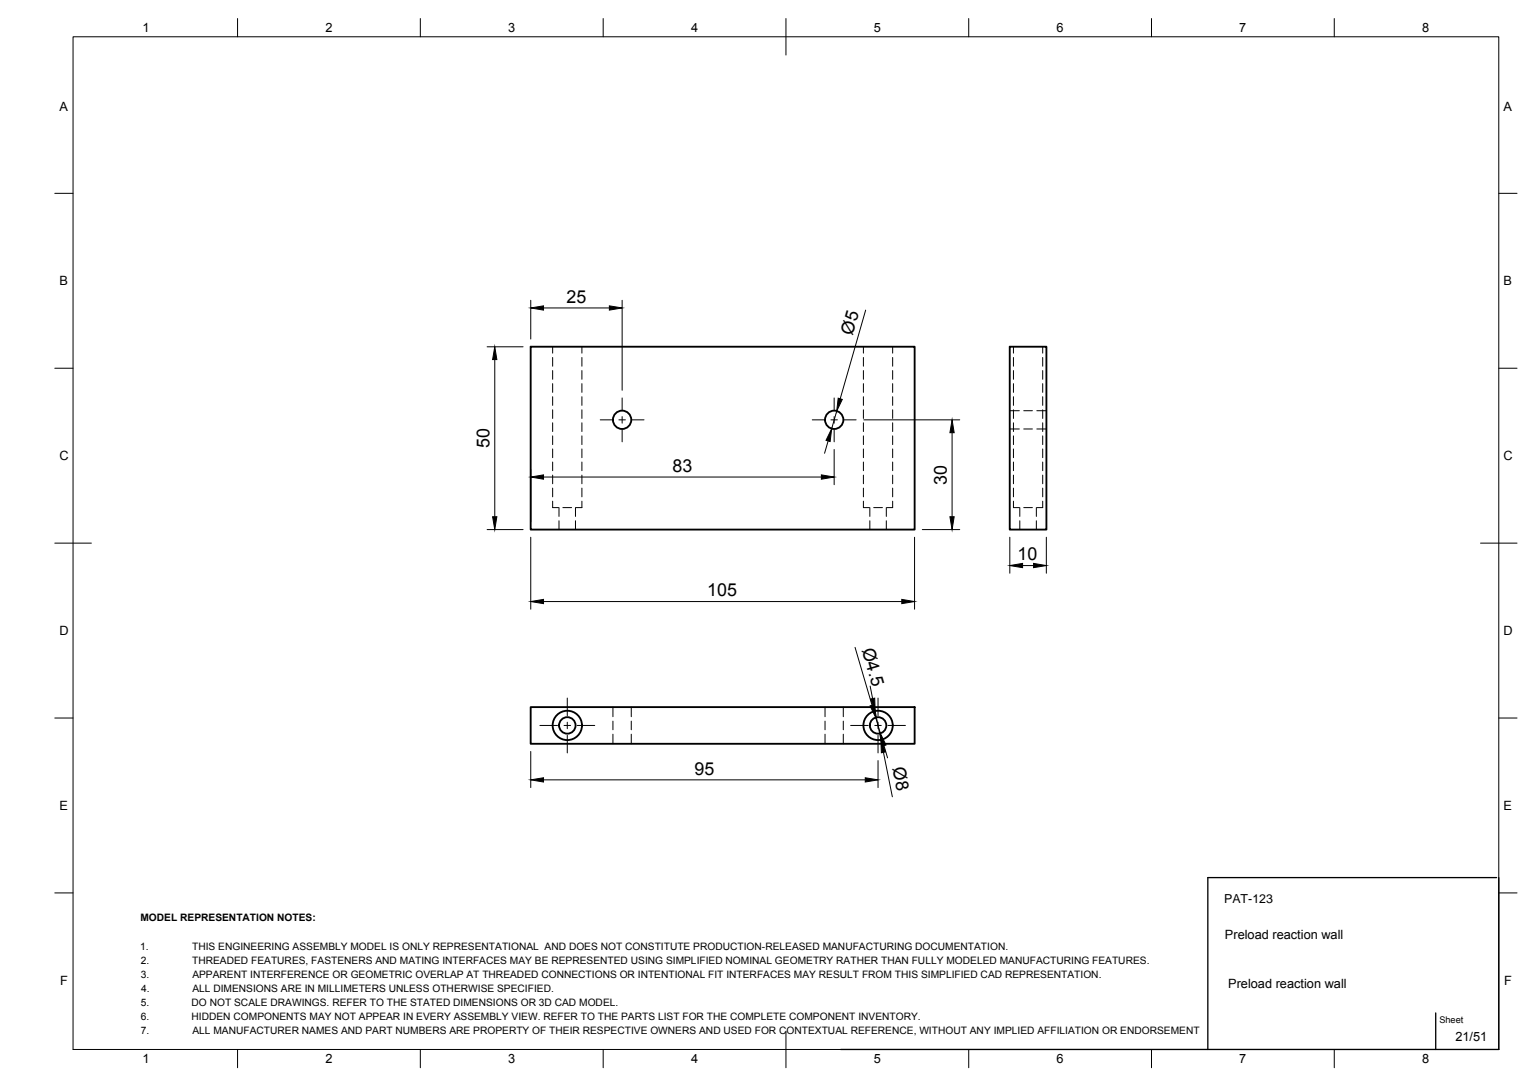
ISO-10303-21;
HEADER;
/* Generated by software containing ST-Developer
 * from STEP Tools, Inc. (www.steptools.com) 
 */

FILE_DESCRIPTION(
/* description */ ('Worm-less right-angle friction wheel drive'),
/* implementation_level */ '2;1');

FILE_NAME(
/* name */ 'Preload reaction wall.step',
/* time_stamp */ '2026-10-28T03:22:36-07:00',
/* author */ (''),
/* organization */ (''),
/* preprocessor_version */ 'ST-DEVELOPER v20.2',
/* originating_system */ 'Autodesk Translation Framework v15.17.0.0',
/* authorisation */ '');

FILE_SCHEMA (('AUTOMOTIVE_DESIGN { 1 0 10303 214 3 1 1 }'));
ENDSEC;

DATA;
#10=MECHANICAL_DESIGN_GEOMETRIC_PRESENTATION_REPRESENTATION('',(#627),#17046);
#533=SHAPE_REPRESENTATION_RELATIONSHIP('SRR','None',#17276,#580);
#580=ADVANCED_BREP_SHAPE_REPRESENTATION('',(#681),#17012);
#627=STYLED_ITEM('',(#17605),#681);
#681=MANIFOLD_SOLID_BREP('Body1',#8182);
#895=FACE_BOUND('',#2060,.T.);
#896=FACE_BOUND('',#2064,.T.);
#897=FACE_BOUND('',#2067,.T.);
#898=FACE_BOUND('',#2068,.T.);
#899=FACE_BOUND('',#2071,.T.);
#900=FACE_BOUND('',#2072,.T.);
#901=FACE_BOUND('',#2075,.T.);
#902=FACE_BOUND('',#2076,.T.);
#903=FACE_BOUND('',#2078,.T.);
#904=FACE_BOUND('',#2079,.T.);
#1048=PLANE('',#9184);
#1049=PLANE('',#9191);
#1050=PLANE('',#9195);
#1051=PLANE('',#9196);
#1052=PLANE('',#9197);
#1053=PLANE('',#9198);
#1054=PLANE('',#9199);
#1055=PLANE('',#9200);
#1410=FACE_OUTER_BOUND('',#2056,.T.);
#1411=FACE_OUTER_BOUND('',#2057,.T.);
#1412=FACE_OUTER_BOUND('',#2058,.T.);
#1413=FACE_OUTER_BOUND('',#2059,.T.);
#1414=FACE_OUTER_BOUND('',#2061,.T.);
#1415=FACE_OUTER_BOUND('',#2062,.T.);
#1416=FACE_OUTER_BOUND('',#2063,.T.);
#1417=FACE_OUTER_BOUND('',#2065,.T.);
#1418=FACE_OUTER_BOUND('',#2066,.T.);
#1419=FACE_OUTER_BOUND('',#2069,.T.);
#1420=FACE_OUTER_BOUND('',#2070,.T.);
#1421=FACE_OUTER_BOUND('',#2073,.T.);
#1422=FACE_OUTER_BOUND('',#2074,.T.);
#1423=FACE_OUTER_BOUND('',#2077,.T.);
#2056=EDGE_LOOP('',(#6506,#6507,#6508,#6509));
#2057=EDGE_LOOP('',(#6510,#6511,#6512,#6513));
#2058=EDGE_LOOP('',(#6514,#6515,#6516,#6517));
#2059=EDGE_LOOP('',(#6518));
#2060=EDGE_LOOP('',(#6519));
#2061=EDGE_LOOP('',(#6520,#6521,#6522,#6523));
#2062=EDGE_LOOP('',(#6524,#6525,#6526,#6527));
#2063=EDGE_LOOP('',(#6528));
#2064=EDGE_LOOP('',(#6529));
#2065=EDGE_LOOP('',(#6530,#6531,#6532,#6533));
#2066=EDGE_LOOP('',(#6534,#6535,#6536,#6537));
#2067=EDGE_LOOP('',(#6538));
#2068=EDGE_LOOP('',(#6539));
#2069=EDGE_LOOP('',(#6540,#6541,#6542,#6543));
#2070=EDGE_LOOP('',(#6544,#6545,#6546,#6547));
#2071=EDGE_LOOP('',(#6548));
#2072=EDGE_LOOP('',(#6549));
#2073=EDGE_LOOP('',(#6550,#6551,#6552,#6553));
#2074=EDGE_LOOP('',(#6554,#6555,#6556,#6557));
#2075=EDGE_LOOP('',(#6558));
#2076=EDGE_LOOP('',(#6559));
#2077=EDGE_LOOP('',(#6560,#6561,#6562,#6563));
#2078=EDGE_LOOP('',(#6564));
#2079=EDGE_LOOP('',(#6565));
#2651=LINE('',#13410,#3191);
#2652=LINE('',#13416,#3192);
#2653=LINE('',#13422,#3193);
#2654=LINE('',#13430,#3194);
#2655=LINE('',#13435,#3195);
#2656=LINE('',#13443,#3196);
#2657=LINE('',#13447,#3197);
#2658=LINE('',#13449,#3198);
#2659=LINE('',#13451,#3199);
#2660=LINE('',#13452,#3200);
#2661=LINE('',#13455,#3201);
#2662=LINE('',#13457,#3202);
#2663=LINE('',#13458,#3203);
#2664=LINE('',#13461,#3204);
#2665=LINE('',#13463,#3205);
#2666=LINE('',#13464,#3206);
#2667=LINE('',#13466,#3207);
#2668=LINE('',#13467,#3208);
#3191=VECTOR('',#10917,0.25);
#3192=VECTOR('',#10924,0.25);
#3193=VECTOR('',#10931,0.4);
#3194=VECTOR('',#10942,0.225);
#3195=VECTOR('',#10947,0.4);
#3196=VECTOR('',#10958,0.225);
#3197=VECTOR('',#10961,1.);
#3198=VECTOR('',#10962,1.);
#3199=VECTOR('',#10963,1.);
#3200=VECTOR('',#10964,1.);
#3201=VECTOR('',#10967,1.);
#3202=VECTOR('',#10968,1.);
#3203=VECTOR('',#10969,1.);
#3204=VECTOR('',#10972,1.);
#3205=VECTOR('',#10973,1.);
#3206=VECTOR('',#10974,1.);
#3207=VECTOR('',#10977,1.);
#3208=VECTOR('',#10978,1.);
#3669=CIRCLE('',#9176,0.25);
#3670=CIRCLE('',#9177,0.25);
#3671=CIRCLE('',#9179,0.25);
#3672=CIRCLE('',#9180,0.25);
#3673=CIRCLE('',#9182,0.4);
#3674=CIRCLE('',#9183,0.4);
#3675=CIRCLE('',#9185,0.225);
#3676=CIRCLE('',#9187,0.225);
#3677=CIRCLE('',#9189,0.4);
#3678=CIRCLE('',#9190,0.4);
#3679=CIRCLE('',#9192,0.225);
#3680=CIRCLE('',#9194,0.225);
#4193=VERTEX_POINT('',#13407);
#4194=VERTEX_POINT('',#13409);
#4195=VERTEX_POINT('',#13413);
#4196=VERTEX_POINT('',#13415);
#4197=VERTEX_POINT('',#13419);
#4198=VERTEX_POINT('',#13421);
#4199=VERTEX_POINT('',#13425);
#4200=VERTEX_POINT('',#13428);
#4201=VERTEX_POINT('',#13432);
#4202=VERTEX_POINT('',#13434);
#4203=VERTEX_POINT('',#13438);
#4204=VERTEX_POINT('',#13441);
#4205=VERTEX_POINT('',#13445);
#4206=VERTEX_POINT('',#13446);
#4207=VERTEX_POINT('',#13448);
#4208=VERTEX_POINT('',#13450);
#4209=VERTEX_POINT('',#13454);
#4210=VERTEX_POINT('',#13456);
#4211=VERTEX_POINT('',#13460);
#4212=VERTEX_POINT('',#13462);
#5022=EDGE_CURVE('',#4193,#4193,#3669,.T.);
#5023=EDGE_CURVE('',#4193,#4194,#2651,.T.);
#5024=EDGE_CURVE('',#4194,#4194,#3670,.T.);
#5025=EDGE_CURVE('',#4195,#4195,#3671,.T.);
#5026=EDGE_CURVE('',#4195,#4196,#2652,.T.);
#5027=EDGE_CURVE('',#4196,#4196,#3672,.T.);
#5028=EDGE_CURVE('',#4197,#4197,#3673,.T.);
#5029=EDGE_CURVE('',#4197,#4198,#2653,.T.);
#5030=EDGE_CURVE('',#4198,#4198,#3674,.T.);
#5031=EDGE_CURVE('',#4199,#4199,#3675,.T.);
#5032=EDGE_CURVE('',#4200,#4200,#3676,.T.);
#5033=EDGE_CURVE('',#4200,#4199,#2654,.T.);
#5034=EDGE_CURVE('',#4201,#4201,#3677,.T.);
#5035=EDGE_CURVE('',#4201,#4202,#2655,.T.);
#5036=EDGE_CURVE('',#4202,#4202,#3678,.T.);
#5037=EDGE_CURVE('',#4203,#4203,#3679,.T.);
#5038=EDGE_CURVE('',#4204,#4204,#3680,.T.);
#5039=EDGE_CURVE('',#4204,#4203,#2656,.T.);
#5040=EDGE_CURVE('',#4205,#4206,#2657,.T.);
#5041=EDGE_CURVE('',#4206,#4207,#2658,.T.);
#5042=EDGE_CURVE('',#4208,#4207,#2659,.T.);
#5043=EDGE_CURVE('',#4205,#4208,#2660,.T.);
#5044=EDGE_CURVE('',#4209,#4205,#2661,.T.);
#5045=EDGE_CURVE('',#4210,#4208,#2662,.T.);
#5046=EDGE_CURVE('',#4209,#4210,#2663,.T.);
#5047=EDGE_CURVE('',#4211,#4209,#2664,.T.);
#5048=EDGE_CURVE('',#4212,#4210,#2665,.T.);
#5049=EDGE_CURVE('',#4211,#4212,#2666,.T.);
#5050=EDGE_CURVE('',#4206,#4211,#2667,.T.);
#5051=EDGE_CURVE('',#4207,#4212,#2668,.T.);
#6506=ORIENTED_EDGE('',*,*,#5022,.F.);
#6507=ORIENTED_EDGE('',*,*,#5023,.T.);
#6508=ORIENTED_EDGE('',*,*,#5024,.F.);
#6509=ORIENTED_EDGE('',*,*,#5023,.F.);
#6510=ORIENTED_EDGE('',*,*,#5025,.F.);
#6511=ORIENTED_EDGE('',*,*,#5026,.T.);
#6512=ORIENTED_EDGE('',*,*,#5027,.F.);
#6513=ORIENTED_EDGE('',*,*,#5026,.F.);
#6514=ORIENTED_EDGE('',*,*,#5028,.F.);
#6515=ORIENTED_EDGE('',*,*,#5029,.T.);
#6516=ORIENTED_EDGE('',*,*,#5030,.F.);
#6517=ORIENTED_EDGE('',*,*,#5029,.F.);
#6518=ORIENTED_EDGE('',*,*,#5028,.T.);
#6519=ORIENTED_EDGE('',*,*,#5031,.F.);
#6520=ORIENTED_EDGE('',*,*,#5032,.F.);
#6521=ORIENTED_EDGE('',*,*,#5033,.T.);
#6522=ORIENTED_EDGE('',*,*,#5031,.T.);
#6523=ORIENTED_EDGE('',*,*,#5033,.F.);
#6524=ORIENTED_EDGE('',*,*,#5034,.F.);
#6525=ORIENTED_EDGE('',*,*,#5035,.T.);
#6526=ORIENTED_EDGE('',*,*,#5036,.F.);
#6527=ORIENTED_EDGE('',*,*,#5035,.F.);
#6528=ORIENTED_EDGE('',*,*,#5034,.T.);
#6529=ORIENTED_EDGE('',*,*,#5037,.F.);
#6530=ORIENTED_EDGE('',*,*,#5038,.F.);
#6531=ORIENTED_EDGE('',*,*,#5039,.T.);
#6532=ORIENTED_EDGE('',*,*,#5037,.T.);
#6533=ORIENTED_EDGE('',*,*,#5039,.F.);
#6534=ORIENTED_EDGE('',*,*,#5040,.T.);
#6535=ORIENTED_EDGE('',*,*,#5041,.T.);
#6536=ORIENTED_EDGE('',*,*,#5042,.F.);
#6537=ORIENTED_EDGE('',*,*,#5043,.F.);
#6538=ORIENTED_EDGE('',*,*,#5024,.T.);
#6539=ORIENTED_EDGE('',*,*,#5027,.T.);
#6540=ORIENTED_EDGE('',*,*,#5044,.T.);
#6541=ORIENTED_EDGE('',*,*,#5043,.T.);
#6542=ORIENTED_EDGE('',*,*,#5045,.F.);
#6543=ORIENTED_EDGE('',*,*,#5046,.F.);
#6544=ORIENTED_EDGE('',*,*,#5047,.T.);
#6545=ORIENTED_EDGE('',*,*,#5046,.T.);
#6546=ORIENTED_EDGE('',*,*,#5048,.F.);
#6547=ORIENTED_EDGE('',*,*,#5049,.F.);
#6548=ORIENTED_EDGE('',*,*,#5022,.T.);
#6549=ORIENTED_EDGE('',*,*,#5025,.T.);
#6550=ORIENTED_EDGE('',*,*,#5050,.T.);
#6551=ORIENTED_EDGE('',*,*,#5049,.T.);
#6552=ORIENTED_EDGE('',*,*,#5051,.F.);
#6553=ORIENTED_EDGE('',*,*,#5041,.F.);
#6554=ORIENTED_EDGE('',*,*,#5051,.T.);
#6555=ORIENTED_EDGE('',*,*,#5048,.T.);
#6556=ORIENTED_EDGE('',*,*,#5045,.T.);
#6557=ORIENTED_EDGE('',*,*,#5042,.T.);
#6558=ORIENTED_EDGE('',*,*,#5030,.T.);
#6559=ORIENTED_EDGE('',*,*,#5036,.T.);
#6560=ORIENTED_EDGE('',*,*,#5050,.F.);
#6561=ORIENTED_EDGE('',*,*,#5040,.F.);
#6562=ORIENTED_EDGE('',*,*,#5044,.F.);
#6563=ORIENTED_EDGE('',*,*,#5047,.F.);
#6564=ORIENTED_EDGE('',*,*,#5032,.T.);
#6565=ORIENTED_EDGE('',*,*,#5038,.T.);
#7636=CYLINDRICAL_SURFACE('',#9175,0.25);
#7637=CYLINDRICAL_SURFACE('',#9178,0.25);
#7638=CYLINDRICAL_SURFACE('',#9181,0.4);
#7639=CYLINDRICAL_SURFACE('',#9186,0.225);
#7640=CYLINDRICAL_SURFACE('',#9188,0.4);
#7641=CYLINDRICAL_SURFACE('',#9193,0.225);
#7902=ADVANCED_FACE('',(#1410),#7636,.F.);
#7903=ADVANCED_FACE('',(#1411),#7637,.F.);
#7904=ADVANCED_FACE('',(#1412),#7638,.F.);
#7905=ADVANCED_FACE('',(#1413,#895),#1048,.T.);
#7906=ADVANCED_FACE('',(#1414),#7639,.F.);
#7907=ADVANCED_FACE('',(#1415),#7640,.F.);
#7908=ADVANCED_FACE('',(#1416,#896),#1049,.T.);
#7909=ADVANCED_FACE('',(#1417),#7641,.F.);
#7910=ADVANCED_FACE('',(#1418,#897,#898),#1050,.T.);
#7911=ADVANCED_FACE('',(#1419),#1051,.T.);
#7912=ADVANCED_FACE('',(#1420,#899,#900),#1052,.T.);
#7913=ADVANCED_FACE('',(#1421),#1053,.T.);
#7914=ADVANCED_FACE('',(#1422,#901,#902),#1054,.T.);
#7915=ADVANCED_FACE('',(#1423,#903,#904),#1055,.F.);
#8182=CLOSED_SHELL('',(#7902,#7903,#7904,#7905,#7906,#7907,#7908,#7909,
#7910,#7911,#7912,#7913,#7914,#7915));
#9174=AXIS2_PLACEMENT_3D('',#13405,#10911,#10912);
#9175=AXIS2_PLACEMENT_3D('',#13406,#10913,#10914);
#9176=AXIS2_PLACEMENT_3D('',#13408,#10915,#10916);
#9177=AXIS2_PLACEMENT_3D('',#13411,#10918,#10919);
#9178=AXIS2_PLACEMENT_3D('',#13412,#10920,#10921);
#9179=AXIS2_PLACEMENT_3D('',#13414,#10922,#10923);
#9180=AXIS2_PLACEMENT_3D('',#13417,#10925,#10926);
#9181=AXIS2_PLACEMENT_3D('',#13418,#10927,#10928);
#9182=AXIS2_PLACEMENT_3D('',#13420,#10929,#10930);
#9183=AXIS2_PLACEMENT_3D('',#13423,#10932,#10933);
#9184=AXIS2_PLACEMENT_3D('',#13424,#10934,#10935);
#9185=AXIS2_PLACEMENT_3D('',#13426,#10936,#10937);
#9186=AXIS2_PLACEMENT_3D('',#13427,#10938,#10939);
#9187=AXIS2_PLACEMENT_3D('',#13429,#10940,#10941);
#9188=AXIS2_PLACEMENT_3D('',#13431,#10943,#10944);
#9189=AXIS2_PLACEMENT_3D('',#13433,#10945,#10946);
#9190=AXIS2_PLACEMENT_3D('',#13436,#10948,#10949);
#9191=AXIS2_PLACEMENT_3D('',#13437,#10950,#10951);
#9192=AXIS2_PLACEMENT_3D('',#13439,#10952,#10953);
#9193=AXIS2_PLACEMENT_3D('',#13440,#10954,#10955);
#9194=AXIS2_PLACEMENT_3D('',#13442,#10956,#10957);
#9195=AXIS2_PLACEMENT_3D('',#13444,#10959,#10960);
#9196=AXIS2_PLACEMENT_3D('',#13453,#10965,#10966);
#9197=AXIS2_PLACEMENT_3D('',#13459,#10970,#10971);
#9198=AXIS2_PLACEMENT_3D('',#13465,#10975,#10976);
#9199=AXIS2_PLACEMENT_3D('',#13468,#10979,#10980);
#9200=AXIS2_PLACEMENT_3D('',#13469,#10981,#10982);
#10911=DIRECTION('axis',(0.,0.,1.));
#10912=DIRECTION('refdir',(1.,0.,0.));
#10913=DIRECTION('center_axis',(0.,1.,0.));
#10914=DIRECTION('ref_axis',(1.,0.,0.));
#10915=DIRECTION('center_axis',(0.,1.,0.));
#10916=DIRECTION('ref_axis',(1.,0.,0.));
#10917=DIRECTION('',(0.,1.,0.));
#10918=DIRECTION('center_axis',(0.,-1.,0.));
#10919=DIRECTION('ref_axis',(1.,0.,0.));
#10920=DIRECTION('center_axis',(0.,1.,0.));
#10921=DIRECTION('ref_axis',(1.,0.,0.));
#10922=DIRECTION('center_axis',(0.,1.,0.));
#10923=DIRECTION('ref_axis',(1.,0.,0.));
#10924=DIRECTION('',(0.,1.,0.));
#10925=DIRECTION('center_axis',(0.,-1.,0.));
#10926=DIRECTION('ref_axis',(1.,0.,0.));
#10927=DIRECTION('center_axis',(0.,0.,1.));
#10928=DIRECTION('ref_axis',(1.,0.,0.));
#10929=DIRECTION('center_axis',(0.,0.,1.));
#10930=DIRECTION('ref_axis',(1.,0.,0.));
#10931=DIRECTION('',(0.,0.,1.));
#10932=DIRECTION('center_axis',(0.,0.,-1.));
#10933=DIRECTION('ref_axis',(1.,0.,0.));
#10934=DIRECTION('center_axis',(0.,0.,1.));
#10935=DIRECTION('ref_axis',(1.,0.,0.));
#10936=DIRECTION('center_axis',(0.,0.,1.));
#10937=DIRECTION('ref_axis',(1.,0.,0.));
#10938=DIRECTION('center_axis',(0.,0.,1.));
#10939=DIRECTION('ref_axis',(1.,0.,0.));
#10940=DIRECTION('center_axis',(0.,0.,1.));
#10941=DIRECTION('ref_axis',(1.,0.,0.));
#10942=DIRECTION('',(0.,0.,1.));
#10943=DIRECTION('center_axis',(0.,0.,1.));
#10944=DIRECTION('ref_axis',(1.,0.,0.));
#10945=DIRECTION('center_axis',(0.,0.,1.));
#10946=DIRECTION('ref_axis',(1.,0.,0.));
#10947=DIRECTION('',(0.,0.,1.));
#10948=DIRECTION('center_axis',(0.,0.,-1.));
#10949=DIRECTION('ref_axis',(1.,0.,0.));
#10950=DIRECTION('center_axis',(0.,0.,1.));
#10951=DIRECTION('ref_axis',(1.,0.,0.));
#10952=DIRECTION('center_axis',(0.,0.,1.));
#10953=DIRECTION('ref_axis',(1.,0.,0.));
#10954=DIRECTION('center_axis',(0.,0.,1.));
#10955=DIRECTION('ref_axis',(1.,0.,0.));
#10956=DIRECTION('center_axis',(0.,0.,1.));
#10957=DIRECTION('ref_axis',(1.,0.,0.));
#10958=DIRECTION('',(0.,0.,1.));
#10959=DIRECTION('center_axis',(0.,1.,0.));
#10960=DIRECTION('ref_axis',(-1.,0.,0.));
#10961=DIRECTION('',(-1.,0.,0.));
#10962=DIRECTION('',(0.,0.,1.));
#10963=DIRECTION('',(-1.,0.,0.));
#10964=DIRECTION('',(0.,0.,1.));
#10965=DIRECTION('center_axis',(1.,0.,0.));
#10966=DIRECTION('ref_axis',(0.,1.,0.));
#10967=DIRECTION('',(0.,1.,0.));
#10968=DIRECTION('',(0.,1.,0.));
#10969=DIRECTION('',(0.,0.,1.));
#10970=DIRECTION('center_axis',(0.,-1.,0.));
#10971=DIRECTION('ref_axis',(1.,0.,0.));
#10972=DIRECTION('',(1.,0.,0.));
#10973=DIRECTION('',(1.,0.,0.));
#10974=DIRECTION('',(0.,0.,1.));
#10975=DIRECTION('center_axis',(-1.,0.,0.));
#10976=DIRECTION('ref_axis',(0.,-1.,0.));
#10977=DIRECTION('',(0.,-1.,0.));
#10978=DIRECTION('',(0.,-1.,0.));
#10979=DIRECTION('center_axis',(0.,0.,1.));
#10980=DIRECTION('ref_axis',(1.,0.,0.));
#10981=DIRECTION('center_axis',(0.,0.,1.));
#10982=DIRECTION('ref_axis',(1.,0.,0.));
#13405=CARTESIAN_POINT('',(0.,0.,0.));
#13406=CARTESIAN_POINT('Origin',(5.5,7.9,4.));
#13407=CARTESIAN_POINT('',(5.25,8.,4.));
#13408=CARTESIAN_POINT('Origin',(5.5,8.,4.));
#13409=CARTESIAN_POINT('',(5.25,9.,4.));
#13410=CARTESIAN_POINT('',(5.25,7.9,4.));
#13411=CARTESIAN_POINT('Origin',(5.5,9.,4.));
#13412=CARTESIAN_POINT('Origin',(-0.3,7.9,4.));
#13413=CARTESIAN_POINT('',(-0.55,8.,4.));
#13414=CARTESIAN_POINT('Origin',(-0.3,8.,4.));
#13415=CARTESIAN_POINT('',(-0.55,9.,4.));
#13416=CARTESIAN_POINT('',(-0.55,7.9,4.));
#13417=CARTESIAN_POINT('Origin',(-0.3,9.,4.));
#13418=CARTESIAN_POINT('Origin',(7.,8.5,1.6));
#13419=CARTESIAN_POINT('',(6.6,8.5,1.6));
#13420=CARTESIAN_POINT('Origin',(7.,8.5,1.6));
#13421=CARTESIAN_POINT('',(6.6,8.5,6.));
#13422=CARTESIAN_POINT('',(6.6,8.5,1.6));
#13423=CARTESIAN_POINT('Origin',(7.,8.5,6.));
#13424=CARTESIAN_POINT('Origin',(7.,8.5,1.6));
#13425=CARTESIAN_POINT('',(6.775,8.5,1.6));
#13426=CARTESIAN_POINT('Origin',(7.,8.5,1.6));
#13427=CARTESIAN_POINT('Origin',(7.,8.5,0.9));
#13428=CARTESIAN_POINT('',(6.775,8.5,1.));
#13429=CARTESIAN_POINT('Origin',(7.,8.5,1.));
#13430=CARTESIAN_POINT('',(6.775,8.5,0.9));
#13431=CARTESIAN_POINT('Origin',(-1.5,8.5,1.6));
#13432=CARTESIAN_POINT('',(-1.9,8.5,1.6));
#13433=CARTESIAN_POINT('Origin',(-1.5,8.5,1.6));
#13434=CARTESIAN_POINT('',(-1.9,8.5,6.));
#13435=CARTESIAN_POINT('',(-1.9,8.5,1.6));
#13436=CARTESIAN_POINT('Origin',(-1.5,8.5,6.));
#13437=CARTESIAN_POINT('Origin',(-1.5,8.5,1.6));
#13438=CARTESIAN_POINT('',(-1.725,8.5,1.6));
#13439=CARTESIAN_POINT('Origin',(-1.5,8.5,1.6));
#13440=CARTESIAN_POINT('Origin',(-1.5,8.5,0.9));
#13441=CARTESIAN_POINT('',(-1.725,8.5,1.));
#13442=CARTESIAN_POINT('Origin',(-1.5,8.5,1.));
#13443=CARTESIAN_POINT('',(-1.725,8.5,0.9));
#13444=CARTESIAN_POINT('Origin',(8.,9.,1.));
#13445=CARTESIAN_POINT('',(8.,9.,1.));
#13446=CARTESIAN_POINT('',(-2.5,9.,1.));
#13447=CARTESIAN_POINT('',(8.,9.,1.));
#13448=CARTESIAN_POINT('',(-2.5,9.,6.));
#13449=CARTESIAN_POINT('',(-2.5,9.,1.));
#13450=CARTESIAN_POINT('',(8.,9.,6.));
#13451=CARTESIAN_POINT('',(8.,9.,6.));
#13452=CARTESIAN_POINT('',(8.,9.,1.));
#13453=CARTESIAN_POINT('Origin',(8.,8.,1.));
#13454=CARTESIAN_POINT('',(8.,8.,1.));
#13455=CARTESIAN_POINT('',(8.,8.,1.));
#13456=CARTESIAN_POINT('',(8.,8.,6.));
#13457=CARTESIAN_POINT('',(8.,8.,6.));
#13458=CARTESIAN_POINT('',(8.,8.,1.));
#13459=CARTESIAN_POINT('Origin',(-2.5,8.,1.));
#13460=CARTESIAN_POINT('',(-2.5,8.,1.));
#13461=CARTESIAN_POINT('',(-2.5,8.,1.));
#13462=CARTESIAN_POINT('',(-2.5,8.,6.));
#13463=CARTESIAN_POINT('',(-2.5,8.,6.));
#13464=CARTESIAN_POINT('',(-2.5,8.,1.));
#13465=CARTESIAN_POINT('Origin',(-2.5,9.,1.));
#13466=CARTESIAN_POINT('',(-2.5,9.,1.));
#13467=CARTESIAN_POINT('',(-2.5,9.,6.));
#13468=CARTESIAN_POINT('Origin',(2.75,8.5,6.));
#13469=CARTESIAN_POINT('Origin',(2.75,8.5,1.));
#16959=UNCERTAINTY_MEASURE_WITH_UNIT(LENGTH_MEASURE(0.001),#17047,
'DISTANCE_ACCURACY_VALUE',
'Maximum model space distance between geometric entities at asserted c
onnectivities');
#16993=UNCERTAINTY_MEASURE_WITH_UNIT(LENGTH_MEASURE(0.001),#17047,
'DISTANCE_ACCURACY_VALUE',
'Maximum model space distance between geometric entities at asserted c
onnectivities');
#17012=(
GEOMETRIC_REPRESENTATION_CONTEXT(3)
GLOBAL_UNCERTAINTY_ASSIGNED_CONTEXT((#16959))
GLOBAL_UNIT_ASSIGNED_CONTEXT((#17047,#17049,#17050))
REPRESENTATION_CONTEXT('','3D')
);
#17046=(
GEOMETRIC_REPRESENTATION_CONTEXT(3)
GLOBAL_UNCERTAINTY_ASSIGNED_CONTEXT((#16993))
GLOBAL_UNIT_ASSIGNED_CONTEXT((#17047,#17049,#17050))
REPRESENTATION_CONTEXT('','3D')
);
#17047=(
LENGTH_UNIT()
NAMED_UNIT(*)
SI_UNIT(.CENTI.,.METRE.)
);
#17049=(
NAMED_UNIT(*)
PLANE_ANGLE_UNIT()
SI_UNIT($,.RADIAN.)
);
#17050=(
NAMED_UNIT(*)
SI_UNIT($,.STERADIAN.)
SOLID_ANGLE_UNIT()
);
#17069=SHAPE_DEFINITION_REPRESENTATION(#17121,#17276);
#17121=PRODUCT_DEFINITION_SHAPE('',$,#17329);
#17276=SHAPE_REPRESENTATION('',(#9174),#17012);
#17310=PRODUCT_DEFINITION_CONTEXT('part definition',#17468,'design');
#17329=PRODUCT_DEFINITION('Preload reaction wall',
'Preload reaction wall',#17381,#17310);
#17381=PRODUCT_DEFINITION_FORMATION('',$,#17488);
#17468=APPLICATION_CONTEXT(
'Core Data for Automotive Mechanical Design Process');
#17469=PRODUCT_CONTEXT('part definition',#17468,'mechanical');
#17488=PRODUCT('Preload reaction wall','Preload reaction wall',
'Preload reaction wall',(#17469));
#17599=COLOUR_RGB('Off White',0.89,0.88,0.83);
#17600=FILL_AREA_STYLE_COLOUR('',#17599);
#17601=FILL_AREA_STYLE('',(#17600));
#17602=SURFACE_STYLE_FILL_AREA(#17601);
#17603=SURFACE_SIDE_STYLE('',(#17602));
#17604=SURFACE_STYLE_USAGE(.BOTH.,#17603);
#17605=PRESENTATION_STYLE_ASSIGNMENT((#17604));
ENDSEC;
END-ISO-10303-21;
